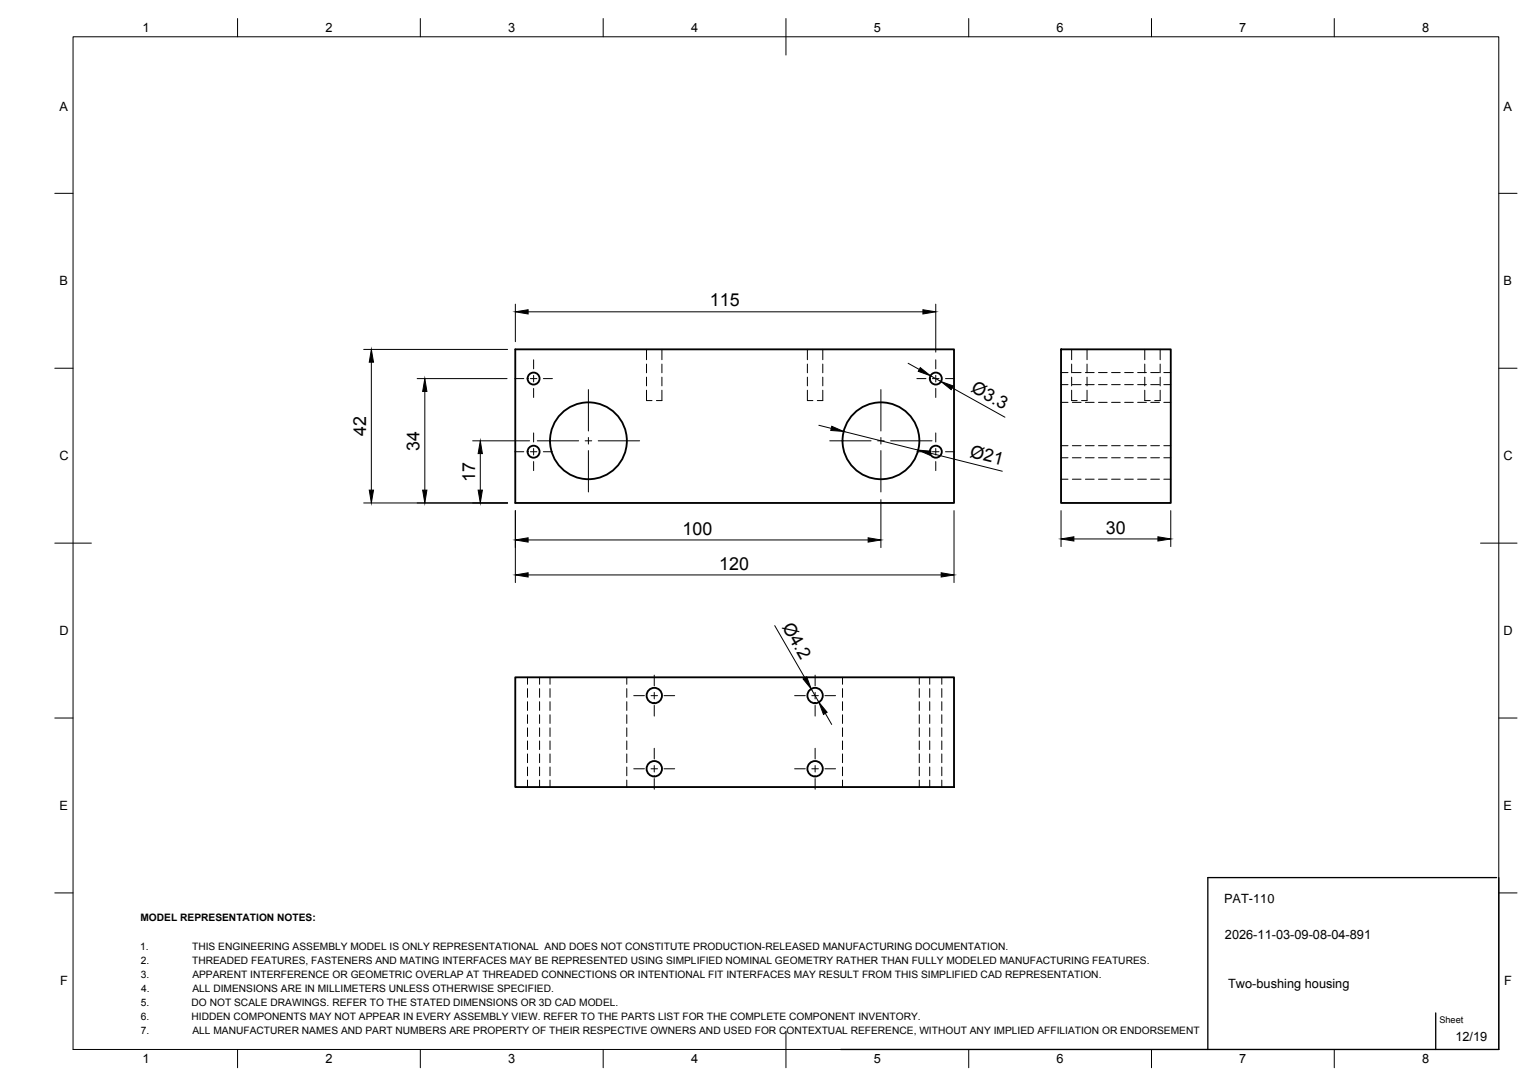
ISO-10303-21;
HEADER;
/* Generated by software containing ST-Developer
 * from STEP Tools, Inc. (www.steptools.com) 
 */

FILE_DESCRIPTION(
/* description */ ('Twin-shaft manual slide'),
/* implementation_level */ '2;1');

FILE_NAME(
/* name */ 'Two-bushing housing.step',
/* time_stamp */ '2026-10-27T18:38:08-07:00',
/* author */ (''),
/* organization */ (''),
/* preprocessor_version */ 'ST-DEVELOPER v20.2',
/* originating_system */ 'Autodesk Translation Framework v15.17.0.0',
/* authorisation */ '');

FILE_SCHEMA (('AUTOMOTIVE_DESIGN { 1 0 10303 214 3 1 1 }'));
ENDSEC;

DATA;
#10=MECHANICAL_DESIGN_GEOMETRIC_PRESENTATION_REPRESENTATION('',(#282),#6463);
#250=SHAPE_REPRESENTATION_RELATIONSHIP('SRR','None',#6569,#266);
#266=ADVANCED_BREP_SHAPE_REPRESENTATION('',(#297),#6452);
#282=STYLED_ITEM('',(#6719),#297);
#297=MANIFOLD_SOLID_BREP('Body1',#3645);
#345=FACE_BOUND('',#870,.T.);
#346=FACE_BOUND('',#871,.T.);
#347=FACE_BOUND('',#872,.T.);
#348=FACE_BOUND('',#873,.T.);
#349=FACE_BOUND('',#874,.T.);
#350=FACE_BOUND('',#875,.T.);
#351=FACE_BOUND('',#878,.T.);
#352=FACE_BOUND('',#879,.T.);
#353=FACE_BOUND('',#880,.T.);
#354=FACE_BOUND('',#881,.T.);
#355=FACE_BOUND('',#882,.T.);
#356=FACE_BOUND('',#883,.T.);
#357=FACE_BOUND('',#885,.T.);
#358=FACE_BOUND('',#886,.T.);
#359=FACE_BOUND('',#887,.T.);
#360=FACE_BOUND('',#888,.T.);
#450=PLANE('',#3997);
#451=PLANE('',#4001);
#452=PLANE('',#4005);
#453=PLANE('',#4009);
#454=PLANE('',#4016);
#455=PLANE('',#4017);
#456=PLANE('',#4018);
#457=PLANE('',#4019);
#458=PLANE('',#4020);
#459=PLANE('',#4021);
#606=FACE_OUTER_BOUND('',#854,.T.);
#607=FACE_OUTER_BOUND('',#855,.T.);
#608=FACE_OUTER_BOUND('',#856,.T.);
#609=FACE_OUTER_BOUND('',#857,.T.);
#610=FACE_OUTER_BOUND('',#858,.T.);
#611=FACE_OUTER_BOUND('',#859,.T.);
#612=FACE_OUTER_BOUND('',#860,.T.);
#613=FACE_OUTER_BOUND('',#861,.T.);
#614=FACE_OUTER_BOUND('',#862,.T.);
#615=FACE_OUTER_BOUND('',#863,.T.);
#616=FACE_OUTER_BOUND('',#864,.T.);
#617=FACE_OUTER_BOUND('',#865,.T.);
#618=FACE_OUTER_BOUND('',#866,.T.);
#619=FACE_OUTER_BOUND('',#867,.T.);
#620=FACE_OUTER_BOUND('',#868,.T.);
#621=FACE_OUTER_BOUND('',#869,.T.);
#622=FACE_OUTER_BOUND('',#876,.T.);
#623=FACE_OUTER_BOUND('',#877,.T.);
#624=FACE_OUTER_BOUND('',#884,.T.);
#625=FACE_OUTER_BOUND('',#889,.T.);
#854=EDGE_LOOP('',(#2856,#2857,#2858,#2859));
#855=EDGE_LOOP('',(#2860,#2861,#2862,#2863));
#856=EDGE_LOOP('',(#2864,#2865,#2866,#2867));
#857=EDGE_LOOP('',(#2868,#2869,#2870,#2871));
#858=EDGE_LOOP('',(#2872,#2873,#2874,#2875));
#859=EDGE_LOOP('',(#2876));
#860=EDGE_LOOP('',(#2877,#2878,#2879,#2880));
#861=EDGE_LOOP('',(#2881));
#862=EDGE_LOOP('',(#2882,#2883,#2884,#2885));
#863=EDGE_LOOP('',(#2886));
#864=EDGE_LOOP('',(#2887,#2888,#2889,#2890));
#865=EDGE_LOOP('',(#2891));
#866=EDGE_LOOP('',(#2892,#2893,#2894,#2895));
#867=EDGE_LOOP('',(#2896,#2897,#2898,#2899));
#868=EDGE_LOOP('',(#2900,#2901,#2902,#2903));
#869=EDGE_LOOP('',(#2904,#2905,#2906,#2907));
#870=EDGE_LOOP('',(#2908));
#871=EDGE_LOOP('',(#2909));
#872=EDGE_LOOP('',(#2910));
#873=EDGE_LOOP('',(#2911));
#874=EDGE_LOOP('',(#2912));
#875=EDGE_LOOP('',(#2913));
#876=EDGE_LOOP('',(#2914,#2915,#2916,#2917));
#877=EDGE_LOOP('',(#2918,#2919,#2920,#2921));
#878=EDGE_LOOP('',(#2922));
#879=EDGE_LOOP('',(#2923));
#880=EDGE_LOOP('',(#2924));
#881=EDGE_LOOP('',(#2925));
#882=EDGE_LOOP('',(#2926));
#883=EDGE_LOOP('',(#2927));
#884=EDGE_LOOP('',(#2928,#2929,#2930,#2931));
#885=EDGE_LOOP('',(#2932));
#886=EDGE_LOOP('',(#2933));
#887=EDGE_LOOP('',(#2934));
#888=EDGE_LOOP('',(#2935));
#889=EDGE_LOOP('',(#2936,#2937,#2938,#2939));
#1164=LINE('',#5816,#1450);
#1165=LINE('',#5822,#1451);
#1166=LINE('',#5828,#1452);
#1167=LINE('',#5834,#1453);
#1168=LINE('',#5840,#1454);
#1169=LINE('',#5847,#1455);
#1170=LINE('',#5854,#1456);
#1171=LINE('',#5861,#1457);
#1172=LINE('',#5868,#1458);
#1173=LINE('',#5874,#1459);
#1174=LINE('',#5879,#1460);
#1175=LINE('',#5881,#1461);
#1176=LINE('',#5883,#1462);
#1177=LINE('',#5884,#1463);
#1178=LINE('',#5887,#1464);
#1179=LINE('',#5889,#1465);
#1180=LINE('',#5890,#1466);
#1181=LINE('',#5893,#1467);
#1182=LINE('',#5895,#1468);
#1183=LINE('',#5896,#1469);
#1184=LINE('',#5898,#1470);
#1185=LINE('',#5899,#1471);
#1450=VECTOR('',#4692,0.165);
#1451=VECTOR('',#4699,0.165);
#1452=VECTOR('',#4706,0.165);
#1453=VECTOR('',#4713,0.165);
#1454=VECTOR('',#4720,0.210000000000001);
#1455=VECTOR('',#4729,0.210000000000001);
#1456=VECTOR('',#4738,0.210000000000001);
#1457=VECTOR('',#4747,0.210000000000001);
#1458=VECTOR('',#4756,1.05);
#1459=VECTOR('',#4763,1.05);
#1460=VECTOR('',#4768,1.);
#1461=VECTOR('',#4769,1.);
#1462=VECTOR('',#4770,1.);
#1463=VECTOR('',#4771,1.);
#1464=VECTOR('',#4774,1.);
#1465=VECTOR('',#4775,1.);
#1466=VECTOR('',#4776,1.);
#1467=VECTOR('',#4779,1.);
#1468=VECTOR('',#4780,1.);
#1469=VECTOR('',#4781,1.);
#1470=VECTOR('',#4784,1.);
#1471=VECTOR('',#4785,1.);
#1666=CIRCLE('',#3983,0.165);
#1667=CIRCLE('',#3984,0.165);
#1668=CIRCLE('',#3986,0.165);
#1669=CIRCLE('',#3987,0.165);
#1670=CIRCLE('',#3989,0.165);
#1671=CIRCLE('',#3990,0.165);
#1672=CIRCLE('',#3992,0.165);
#1673=CIRCLE('',#3993,0.165);
#1674=CIRCLE('',#3995,0.210000000000001);
#1675=CIRCLE('',#3996,0.210000000000001);
#1676=CIRCLE('',#3999,0.210000000000001);
#1677=CIRCLE('',#4000,0.210000000000001);
#1678=CIRCLE('',#4003,0.210000000000001);
#1679=CIRCLE('',#4004,0.210000000000001);
#1680=CIRCLE('',#4007,0.210000000000001);
#1681=CIRCLE('',#4008,0.210000000000001);
#1682=CIRCLE('',#4011,1.05);
#1683=CIRCLE('',#4012,1.05);
#1684=CIRCLE('',#4014,1.05);
#1685=CIRCLE('',#4015,1.05);
#1883=VERTEX_POINT('',#5813);
#1884=VERTEX_POINT('',#5815);
#1885=VERTEX_POINT('',#5819);
#1886=VERTEX_POINT('',#5821);
#1887=VERTEX_POINT('',#5825);
#1888=VERTEX_POINT('',#5827);
#1889=VERTEX_POINT('',#5831);
#1890=VERTEX_POINT('',#5833);
#1891=VERTEX_POINT('',#5837);
#1892=VERTEX_POINT('',#5839);
#1893=VERTEX_POINT('',#5844);
#1894=VERTEX_POINT('',#5846);
#1895=VERTEX_POINT('',#5851);
#1896=VERTEX_POINT('',#5853);
#1897=VERTEX_POINT('',#5858);
#1898=VERTEX_POINT('',#5860);
#1899=VERTEX_POINT('',#5865);
#1900=VERTEX_POINT('',#5867);
#1901=VERTEX_POINT('',#5871);
#1902=VERTEX_POINT('',#5873);
#1903=VERTEX_POINT('',#5877);
#1904=VERTEX_POINT('',#5878);
#1905=VERTEX_POINT('',#5880);
#1906=VERTEX_POINT('',#5882);
#1907=VERTEX_POINT('',#5886);
#1908=VERTEX_POINT('',#5888);
#1909=VERTEX_POINT('',#5892);
#1910=VERTEX_POINT('',#5894);
#2233=EDGE_CURVE('',#1883,#1883,#1666,.T.);
#2234=EDGE_CURVE('',#1883,#1884,#1164,.T.);
#2235=EDGE_CURVE('',#1884,#1884,#1667,.T.);
#2236=EDGE_CURVE('',#1885,#1885,#1668,.T.);
#2237=EDGE_CURVE('',#1885,#1886,#1165,.T.);
#2238=EDGE_CURVE('',#1886,#1886,#1669,.T.);
#2239=EDGE_CURVE('',#1887,#1887,#1670,.T.);
#2240=EDGE_CURVE('',#1887,#1888,#1166,.T.);
#2241=EDGE_CURVE('',#1888,#1888,#1671,.T.);
#2242=EDGE_CURVE('',#1889,#1889,#1672,.T.);
#2243=EDGE_CURVE('',#1889,#1890,#1167,.T.);
#2244=EDGE_CURVE('',#1890,#1890,#1673,.T.);
#2245=EDGE_CURVE('',#1891,#1891,#1674,.T.);
#2246=EDGE_CURVE('',#1891,#1892,#1168,.T.);
#2247=EDGE_CURVE('',#1892,#1892,#1675,.T.);
#2248=EDGE_CURVE('',#1893,#1893,#1676,.T.);
#2249=EDGE_CURVE('',#1893,#1894,#1169,.T.);
#2250=EDGE_CURVE('',#1894,#1894,#1677,.T.);
#2251=EDGE_CURVE('',#1895,#1895,#1678,.T.);
#2252=EDGE_CURVE('',#1895,#1896,#1170,.T.);
#2253=EDGE_CURVE('',#1896,#1896,#1679,.T.);
#2254=EDGE_CURVE('',#1897,#1897,#1680,.T.);
#2255=EDGE_CURVE('',#1897,#1898,#1171,.T.);
#2256=EDGE_CURVE('',#1898,#1898,#1681,.T.);
#2257=EDGE_CURVE('',#1899,#1899,#1682,.T.);
#2258=EDGE_CURVE('',#1899,#1900,#1172,.T.);
#2259=EDGE_CURVE('',#1900,#1900,#1683,.T.);
#2260=EDGE_CURVE('',#1901,#1901,#1684,.T.);
#2261=EDGE_CURVE('',#1901,#1902,#1173,.T.);
#2262=EDGE_CURVE('',#1902,#1902,#1685,.T.);
#2263=EDGE_CURVE('',#1903,#1904,#1174,.T.);
#2264=EDGE_CURVE('',#1904,#1905,#1175,.T.);
#2265=EDGE_CURVE('',#1906,#1905,#1176,.T.);
#2266=EDGE_CURVE('',#1903,#1906,#1177,.T.);
#2267=EDGE_CURVE('',#1907,#1903,#1178,.T.);
#2268=EDGE_CURVE('',#1908,#1906,#1179,.T.);
#2269=EDGE_CURVE('',#1907,#1908,#1180,.T.);
#2270=EDGE_CURVE('',#1909,#1907,#1181,.T.);
#2271=EDGE_CURVE('',#1910,#1908,#1182,.T.);
#2272=EDGE_CURVE('',#1909,#1910,#1183,.T.);
#2273=EDGE_CURVE('',#1904,#1909,#1184,.T.);
#2274=EDGE_CURVE('',#1905,#1910,#1185,.T.);
#2856=ORIENTED_EDGE('',*,*,#2233,.F.);
#2857=ORIENTED_EDGE('',*,*,#2234,.T.);
#2858=ORIENTED_EDGE('',*,*,#2235,.F.);
#2859=ORIENTED_EDGE('',*,*,#2234,.F.);
#2860=ORIENTED_EDGE('',*,*,#2236,.F.);
#2861=ORIENTED_EDGE('',*,*,#2237,.T.);
#2862=ORIENTED_EDGE('',*,*,#2238,.F.);
#2863=ORIENTED_EDGE('',*,*,#2237,.F.);
#2864=ORIENTED_EDGE('',*,*,#2239,.F.);
#2865=ORIENTED_EDGE('',*,*,#2240,.T.);
#2866=ORIENTED_EDGE('',*,*,#2241,.F.);
#2867=ORIENTED_EDGE('',*,*,#2240,.F.);
#2868=ORIENTED_EDGE('',*,*,#2242,.F.);
#2869=ORIENTED_EDGE('',*,*,#2243,.T.);
#2870=ORIENTED_EDGE('',*,*,#2244,.F.);
#2871=ORIENTED_EDGE('',*,*,#2243,.F.);
#2872=ORIENTED_EDGE('',*,*,#2245,.F.);
#2873=ORIENTED_EDGE('',*,*,#2246,.T.);
#2874=ORIENTED_EDGE('',*,*,#2247,.F.);
#2875=ORIENTED_EDGE('',*,*,#2246,.F.);
#2876=ORIENTED_EDGE('',*,*,#2245,.T.);
#2877=ORIENTED_EDGE('',*,*,#2248,.F.);
#2878=ORIENTED_EDGE('',*,*,#2249,.T.);
#2879=ORIENTED_EDGE('',*,*,#2250,.F.);
#2880=ORIENTED_EDGE('',*,*,#2249,.F.);
#2881=ORIENTED_EDGE('',*,*,#2248,.T.);
#2882=ORIENTED_EDGE('',*,*,#2251,.F.);
#2883=ORIENTED_EDGE('',*,*,#2252,.T.);
#2884=ORIENTED_EDGE('',*,*,#2253,.F.);
#2885=ORIENTED_EDGE('',*,*,#2252,.F.);
#2886=ORIENTED_EDGE('',*,*,#2251,.T.);
#2887=ORIENTED_EDGE('',*,*,#2254,.F.);
#2888=ORIENTED_EDGE('',*,*,#2255,.T.);
#2889=ORIENTED_EDGE('',*,*,#2256,.F.);
#2890=ORIENTED_EDGE('',*,*,#2255,.F.);
#2891=ORIENTED_EDGE('',*,*,#2254,.T.);
#2892=ORIENTED_EDGE('',*,*,#2257,.F.);
#2893=ORIENTED_EDGE('',*,*,#2258,.T.);
#2894=ORIENTED_EDGE('',*,*,#2259,.F.);
#2895=ORIENTED_EDGE('',*,*,#2258,.F.);
#2896=ORIENTED_EDGE('',*,*,#2260,.F.);
#2897=ORIENTED_EDGE('',*,*,#2261,.T.);
#2898=ORIENTED_EDGE('',*,*,#2262,.F.);
#2899=ORIENTED_EDGE('',*,*,#2261,.F.);
#2900=ORIENTED_EDGE('',*,*,#2263,.T.);
#2901=ORIENTED_EDGE('',*,*,#2264,.T.);
#2902=ORIENTED_EDGE('',*,*,#2265,.F.);
#2903=ORIENTED_EDGE('',*,*,#2266,.F.);
#2904=ORIENTED_EDGE('',*,*,#2267,.T.);
#2905=ORIENTED_EDGE('',*,*,#2266,.T.);
#2906=ORIENTED_EDGE('',*,*,#2268,.F.);
#2907=ORIENTED_EDGE('',*,*,#2269,.F.);
#2908=ORIENTED_EDGE('',*,*,#2262,.T.);
#2909=ORIENTED_EDGE('',*,*,#2259,.T.);
#2910=ORIENTED_EDGE('',*,*,#2244,.T.);
#2911=ORIENTED_EDGE('',*,*,#2241,.T.);
#2912=ORIENTED_EDGE('',*,*,#2238,.T.);
#2913=ORIENTED_EDGE('',*,*,#2235,.T.);
#2914=ORIENTED_EDGE('',*,*,#2270,.T.);
#2915=ORIENTED_EDGE('',*,*,#2269,.T.);
#2916=ORIENTED_EDGE('',*,*,#2271,.F.);
#2917=ORIENTED_EDGE('',*,*,#2272,.F.);
#2918=ORIENTED_EDGE('',*,*,#2273,.T.);
#2919=ORIENTED_EDGE('',*,*,#2272,.T.);
#2920=ORIENTED_EDGE('',*,*,#2274,.F.);
#2921=ORIENTED_EDGE('',*,*,#2264,.F.);
#2922=ORIENTED_EDGE('',*,*,#2260,.T.);
#2923=ORIENTED_EDGE('',*,*,#2257,.T.);
#2924=ORIENTED_EDGE('',*,*,#2242,.T.);
#2925=ORIENTED_EDGE('',*,*,#2239,.T.);
#2926=ORIENTED_EDGE('',*,*,#2236,.T.);
#2927=ORIENTED_EDGE('',*,*,#2233,.T.);
#2928=ORIENTED_EDGE('',*,*,#2274,.T.);
#2929=ORIENTED_EDGE('',*,*,#2271,.T.);
#2930=ORIENTED_EDGE('',*,*,#2268,.T.);
#2931=ORIENTED_EDGE('',*,*,#2265,.T.);
#2932=ORIENTED_EDGE('',*,*,#2247,.T.);
#2933=ORIENTED_EDGE('',*,*,#2250,.T.);
#2934=ORIENTED_EDGE('',*,*,#2253,.T.);
#2935=ORIENTED_EDGE('',*,*,#2256,.T.);
#2936=ORIENTED_EDGE('',*,*,#2273,.F.);
#2937=ORIENTED_EDGE('',*,*,#2263,.F.);
#2938=ORIENTED_EDGE('',*,*,#2267,.F.);
#2939=ORIENTED_EDGE('',*,*,#2270,.F.);
#3392=CYLINDRICAL_SURFACE('',#3982,0.165);
#3393=CYLINDRICAL_SURFACE('',#3985,0.165);
#3394=CYLINDRICAL_SURFACE('',#3988,0.165);
#3395=CYLINDRICAL_SURFACE('',#3991,0.165);
#3396=CYLINDRICAL_SURFACE('',#3994,0.210000000000001);
#3397=CYLINDRICAL_SURFACE('',#3998,0.210000000000001);
#3398=CYLINDRICAL_SURFACE('',#4002,0.210000000000001);
#3399=CYLINDRICAL_SURFACE('',#4006,0.210000000000001);
#3400=CYLINDRICAL_SURFACE('',#4010,1.05);
#3401=CYLINDRICAL_SURFACE('',#4013,1.05);
#3511=ADVANCED_FACE('',(#606),#3392,.F.);
#3512=ADVANCED_FACE('',(#607),#3393,.F.);
#3513=ADVANCED_FACE('',(#608),#3394,.F.);
#3514=ADVANCED_FACE('',(#609),#3395,.F.);
#3515=ADVANCED_FACE('',(#610),#3396,.F.);
#3516=ADVANCED_FACE('',(#611),#450,.T.);
#3517=ADVANCED_FACE('',(#612),#3397,.F.);
#3518=ADVANCED_FACE('',(#613),#451,.T.);
#3519=ADVANCED_FACE('',(#614),#3398,.F.);
#3520=ADVANCED_FACE('',(#615),#452,.T.);
#3521=ADVANCED_FACE('',(#616),#3399,.F.);
#3522=ADVANCED_FACE('',(#617),#453,.T.);
#3523=ADVANCED_FACE('',(#618),#3400,.F.);
#3524=ADVANCED_FACE('',(#619),#3401,.F.);
#3525=ADVANCED_FACE('',(#620),#454,.T.);
#3526=ADVANCED_FACE('',(#621,#345,#346,#347,#348,#349,#350),#455,.T.);
#3527=ADVANCED_FACE('',(#622),#456,.T.);
#3528=ADVANCED_FACE('',(#623,#351,#352,#353,#354,#355,#356),#457,.T.);
#3529=ADVANCED_FACE('',(#624,#357,#358,#359,#360),#458,.T.);
#3530=ADVANCED_FACE('',(#625),#459,.F.);
#3645=CLOSED_SHELL('',(#3511,#3512,#3513,#3514,#3515,#3516,#3517,#3518,
#3519,#3520,#3521,#3522,#3523,#3524,#3525,#3526,#3527,#3528,#3529,#3530));
#3981=AXIS2_PLACEMENT_3D('',#5811,#4686,#4687);
#3982=AXIS2_PLACEMENT_3D('',#5812,#4688,#4689);
#3983=AXIS2_PLACEMENT_3D('',#5814,#4690,#4691);
#3984=AXIS2_PLACEMENT_3D('',#5817,#4693,#4694);
#3985=AXIS2_PLACEMENT_3D('',#5818,#4695,#4696);
#3986=AXIS2_PLACEMENT_3D('',#5820,#4697,#4698);
#3987=AXIS2_PLACEMENT_3D('',#5823,#4700,#4701);
#3988=AXIS2_PLACEMENT_3D('',#5824,#4702,#4703);
#3989=AXIS2_PLACEMENT_3D('',#5826,#4704,#4705);
#3990=AXIS2_PLACEMENT_3D('',#5829,#4707,#4708);
#3991=AXIS2_PLACEMENT_3D('',#5830,#4709,#4710);
#3992=AXIS2_PLACEMENT_3D('',#5832,#4711,#4712);
#3993=AXIS2_PLACEMENT_3D('',#5835,#4714,#4715);
#3994=AXIS2_PLACEMENT_3D('',#5836,#4716,#4717);
#3995=AXIS2_PLACEMENT_3D('',#5838,#4718,#4719);
#3996=AXIS2_PLACEMENT_3D('',#5841,#4721,#4722);
#3997=AXIS2_PLACEMENT_3D('',#5842,#4723,#4724);
#3998=AXIS2_PLACEMENT_3D('',#5843,#4725,#4726);
#3999=AXIS2_PLACEMENT_3D('',#5845,#4727,#4728);
#4000=AXIS2_PLACEMENT_3D('',#5848,#4730,#4731);
#4001=AXIS2_PLACEMENT_3D('',#5849,#4732,#4733);
#4002=AXIS2_PLACEMENT_3D('',#5850,#4734,#4735);
#4003=AXIS2_PLACEMENT_3D('',#5852,#4736,#4737);
#4004=AXIS2_PLACEMENT_3D('',#5855,#4739,#4740);
#4005=AXIS2_PLACEMENT_3D('',#5856,#4741,#4742);
#4006=AXIS2_PLACEMENT_3D('',#5857,#4743,#4744);
#4007=AXIS2_PLACEMENT_3D('',#5859,#4745,#4746);
#4008=AXIS2_PLACEMENT_3D('',#5862,#4748,#4749);
#4009=AXIS2_PLACEMENT_3D('',#5863,#4750,#4751);
#4010=AXIS2_PLACEMENT_3D('',#5864,#4752,#4753);
#4011=AXIS2_PLACEMENT_3D('',#5866,#4754,#4755);
#4012=AXIS2_PLACEMENT_3D('',#5869,#4757,#4758);
#4013=AXIS2_PLACEMENT_3D('',#5870,#4759,#4760);
#4014=AXIS2_PLACEMENT_3D('',#5872,#4761,#4762);
#4015=AXIS2_PLACEMENT_3D('',#5875,#4764,#4765);
#4016=AXIS2_PLACEMENT_3D('',#5876,#4766,#4767);
#4017=AXIS2_PLACEMENT_3D('',#5885,#4772,#4773);
#4018=AXIS2_PLACEMENT_3D('',#5891,#4777,#4778);
#4019=AXIS2_PLACEMENT_3D('',#5897,#4782,#4783);
#4020=AXIS2_PLACEMENT_3D('',#5900,#4786,#4787);
#4021=AXIS2_PLACEMENT_3D('',#5901,#4788,#4789);
#4686=DIRECTION('axis',(0.,0.,1.));
#4687=DIRECTION('refdir',(1.,0.,0.));
#4688=DIRECTION('center_axis',(1.,0.,0.));
#4689=DIRECTION('ref_axis',(0.,0.,-1.));
#4690=DIRECTION('center_axis',(1.,0.,0.));
#4691=DIRECTION('ref_axis',(0.,0.,-1.));
#4692=DIRECTION('',(1.,0.,0.));
#4693=DIRECTION('center_axis',(-1.,0.,0.));
#4694=DIRECTION('ref_axis',(0.,0.,-1.));
#4695=DIRECTION('center_axis',(1.,0.,0.));
#4696=DIRECTION('ref_axis',(0.,0.,-1.));
#4697=DIRECTION('center_axis',(1.,0.,0.));
#4698=DIRECTION('ref_axis',(0.,0.,-1.));
#4699=DIRECTION('',(1.,0.,0.));
#4700=DIRECTION('center_axis',(-1.,0.,0.));
#4701=DIRECTION('ref_axis',(0.,0.,-1.));
#4702=DIRECTION('center_axis',(1.,0.,0.));
#4703=DIRECTION('ref_axis',(0.,0.,-1.));
#4704=DIRECTION('center_axis',(1.,0.,0.));
#4705=DIRECTION('ref_axis',(0.,0.,-1.));
#4706=DIRECTION('',(1.,0.,0.));
#4707=DIRECTION('center_axis',(-1.,0.,0.));
#4708=DIRECTION('ref_axis',(0.,0.,-1.));
#4709=DIRECTION('center_axis',(1.,0.,0.));
#4710=DIRECTION('ref_axis',(0.,0.,-1.));
#4711=DIRECTION('center_axis',(1.,0.,0.));
#4712=DIRECTION('ref_axis',(0.,0.,-1.));
#4713=DIRECTION('',(1.,0.,0.));
#4714=DIRECTION('center_axis',(-1.,0.,0.));
#4715=DIRECTION('ref_axis',(0.,0.,-1.));
#4716=DIRECTION('center_axis',(0.,0.,1.));
#4717=DIRECTION('ref_axis',(1.,0.,0.));
#4718=DIRECTION('center_axis',(0.,0.,1.));
#4719=DIRECTION('ref_axis',(1.,0.,0.));
#4720=DIRECTION('',(0.,0.,1.));
#4721=DIRECTION('center_axis',(0.,0.,-1.));
#4722=DIRECTION('ref_axis',(1.,0.,0.));
#4723=DIRECTION('center_axis',(0.,0.,1.));
#4724=DIRECTION('ref_axis',(1.,0.,0.));
#4725=DIRECTION('center_axis',(0.,0.,1.));
#4726=DIRECTION('ref_axis',(1.,0.,0.));
#4727=DIRECTION('center_axis',(0.,0.,1.));
#4728=DIRECTION('ref_axis',(1.,0.,0.));
#4729=DIRECTION('',(0.,0.,1.));
#4730=DIRECTION('center_axis',(0.,0.,-1.));
#4731=DIRECTION('ref_axis',(1.,0.,0.));
#4732=DIRECTION('center_axis',(0.,0.,1.));
#4733=DIRECTION('ref_axis',(1.,0.,0.));
#4734=DIRECTION('center_axis',(0.,0.,1.));
#4735=DIRECTION('ref_axis',(1.,0.,0.));
#4736=DIRECTION('center_axis',(0.,0.,1.));
#4737=DIRECTION('ref_axis',(1.,0.,0.));
#4738=DIRECTION('',(0.,0.,1.));
#4739=DIRECTION('center_axis',(0.,0.,-1.));
#4740=DIRECTION('ref_axis',(1.,0.,0.));
#4741=DIRECTION('center_axis',(0.,0.,1.));
#4742=DIRECTION('ref_axis',(1.,0.,0.));
#4743=DIRECTION('center_axis',(0.,0.,1.));
#4744=DIRECTION('ref_axis',(1.,0.,0.));
#4745=DIRECTION('center_axis',(0.,0.,1.));
#4746=DIRECTION('ref_axis',(1.,0.,0.));
#4747=DIRECTION('',(0.,0.,1.));
#4748=DIRECTION('center_axis',(0.,0.,-1.));
#4749=DIRECTION('ref_axis',(1.,0.,0.));
#4750=DIRECTION('center_axis',(0.,0.,1.));
#4751=DIRECTION('ref_axis',(1.,0.,0.));
#4752=DIRECTION('center_axis',(1.,0.,0.));
#4753=DIRECTION('ref_axis',(0.,0.,-1.));
#4754=DIRECTION('center_axis',(1.,0.,0.));
#4755=DIRECTION('ref_axis',(0.,0.,-1.));
#4756=DIRECTION('',(1.,0.,0.));
#4757=DIRECTION('center_axis',(-1.,0.,0.));
#4758=DIRECTION('ref_axis',(0.,0.,-1.));
#4759=DIRECTION('center_axis',(1.,0.,0.));
#4760=DIRECTION('ref_axis',(0.,0.,-1.));
#4761=DIRECTION('center_axis',(1.,0.,0.));
#4762=DIRECTION('ref_axis',(0.,0.,-1.));
#4763=DIRECTION('',(1.,0.,0.));
#4764=DIRECTION('center_axis',(-1.,0.,0.));
#4765=DIRECTION('ref_axis',(0.,0.,-1.));
#4766=DIRECTION('center_axis',(0.,1.,0.));
#4767=DIRECTION('ref_axis',(-1.,0.,0.));
#4768=DIRECTION('',(-1.,0.,0.));
#4769=DIRECTION('',(0.,0.,1.));
#4770=DIRECTION('',(-1.,0.,0.));
#4771=DIRECTION('',(0.,0.,1.));
#4772=DIRECTION('center_axis',(1.,0.,0.));
#4773=DIRECTION('ref_axis',(0.,1.,0.));
#4774=DIRECTION('',(0.,1.,0.));
#4775=DIRECTION('',(0.,1.,0.));
#4776=DIRECTION('',(0.,0.,1.));
#4777=DIRECTION('center_axis',(0.,-1.,0.));
#4778=DIRECTION('ref_axis',(1.,0.,0.));
#4779=DIRECTION('',(1.,0.,0.));
#4780=DIRECTION('',(1.,0.,0.));
#4781=DIRECTION('',(0.,0.,1.));
#4782=DIRECTION('center_axis',(-1.,0.,0.));
#4783=DIRECTION('ref_axis',(0.,-1.,0.));
#4784=DIRECTION('',(0.,-1.,0.));
#4785=DIRECTION('',(0.,-1.,0.));
#4786=DIRECTION('center_axis',(0.,0.,1.));
#4787=DIRECTION('ref_axis',(1.,0.,0.));
#4788=DIRECTION('center_axis',(0.,0.,1.));
#4789=DIRECTION('ref_axis',(1.,0.,0.));
#5811=CARTESIAN_POINT('',(0.,0.,0.));
#5812=CARTESIAN_POINT('Origin',(13.4,5.5,3.));
#5813=CARTESIAN_POINT('',(13.5,5.5,3.165));
#5814=CARTESIAN_POINT('Origin',(13.5,5.5,3.));
#5815=CARTESIAN_POINT('',(16.5,5.5,3.165));
#5816=CARTESIAN_POINT('',(13.4,5.5,3.165));
#5817=CARTESIAN_POINT('Origin',(16.5,5.5,3.));
#5818=CARTESIAN_POINT('Origin',(13.4,-5.5,5.));
#5819=CARTESIAN_POINT('',(13.5,-5.5,5.165));
#5820=CARTESIAN_POINT('Origin',(13.5,-5.5,5.));
#5821=CARTESIAN_POINT('',(16.5,-5.5,5.165));
#5822=CARTESIAN_POINT('',(13.4,-5.5,5.165));
#5823=CARTESIAN_POINT('Origin',(16.5,-5.5,5.));
#5824=CARTESIAN_POINT('Origin',(13.4,-5.5,3.));
#5825=CARTESIAN_POINT('',(13.5,-5.5,3.165));
#5826=CARTESIAN_POINT('Origin',(13.5,-5.5,3.));
#5827=CARTESIAN_POINT('',(16.5,-5.5,3.165));
#5828=CARTESIAN_POINT('',(13.4,-5.5,3.165));
#5829=CARTESIAN_POINT('Origin',(16.5,-5.5,3.));
#5830=CARTESIAN_POINT('Origin',(13.4,5.5,5.));
#5831=CARTESIAN_POINT('',(13.5,5.5,5.165));
#5832=CARTESIAN_POINT('Origin',(13.5,5.5,5.));
#5833=CARTESIAN_POINT('',(16.5,5.5,5.165));
#5834=CARTESIAN_POINT('',(13.4,5.5,5.165));
#5835=CARTESIAN_POINT('Origin',(16.5,5.5,5.));
#5836=CARTESIAN_POINT('Origin',(16.,-2.2,4.4));
#5837=CARTESIAN_POINT('',(15.79,-2.2,4.4));
#5838=CARTESIAN_POINT('Origin',(16.,-2.2,4.4));
#5839=CARTESIAN_POINT('',(15.79,-2.2,5.8));
#5840=CARTESIAN_POINT('',(15.79,-2.2,4.4));
#5841=CARTESIAN_POINT('Origin',(16.,-2.2,5.8));
#5842=CARTESIAN_POINT('Origin',(16.,-2.2,4.4));
#5843=CARTESIAN_POINT('Origin',(14.,2.2,4.4));
#5844=CARTESIAN_POINT('',(13.79,2.2,4.4));
#5845=CARTESIAN_POINT('Origin',(14.,2.2,4.4));
#5846=CARTESIAN_POINT('',(13.79,2.2,5.8));
#5847=CARTESIAN_POINT('',(13.79,2.2,4.4));
#5848=CARTESIAN_POINT('Origin',(14.,2.2,5.8));
#5849=CARTESIAN_POINT('Origin',(14.,2.2,4.4));
#5850=CARTESIAN_POINT('Origin',(14.,-2.2,4.4));
#5851=CARTESIAN_POINT('',(13.79,-2.2,4.4));
#5852=CARTESIAN_POINT('Origin',(14.,-2.2,4.4));
#5853=CARTESIAN_POINT('',(13.79,-2.2,5.8));
#5854=CARTESIAN_POINT('',(13.79,-2.2,4.4));
#5855=CARTESIAN_POINT('Origin',(14.,-2.2,5.8));
#5856=CARTESIAN_POINT('Origin',(14.,-2.2,4.4));
#5857=CARTESIAN_POINT('Origin',(16.,2.2,4.4));
#5858=CARTESIAN_POINT('',(15.79,2.2,4.4));
#5859=CARTESIAN_POINT('Origin',(16.,2.2,4.4));
#5860=CARTESIAN_POINT('',(15.79,2.2,5.8));
#5861=CARTESIAN_POINT('',(15.79,2.2,4.4));
#5862=CARTESIAN_POINT('Origin',(16.,2.2,5.8));
#5863=CARTESIAN_POINT('Origin',(16.,2.2,4.4));
#5864=CARTESIAN_POINT('Origin',(13.4,-4.,3.3));
#5865=CARTESIAN_POINT('',(13.5,-4.,4.35));
#5866=CARTESIAN_POINT('Origin',(13.5,-4.,3.3));
#5867=CARTESIAN_POINT('',(16.5,-4.,4.35));
#5868=CARTESIAN_POINT('',(13.4,-4.,4.35));
#5869=CARTESIAN_POINT('Origin',(16.5,-4.,3.3));
#5870=CARTESIAN_POINT('Origin',(13.4,4.,3.3));
#5871=CARTESIAN_POINT('',(13.5,4.,4.35));
#5872=CARTESIAN_POINT('Origin',(13.5,4.,3.3));
#5873=CARTESIAN_POINT('',(16.5,4.,4.35));
#5874=CARTESIAN_POINT('',(13.4,4.,4.35));
#5875=CARTESIAN_POINT('Origin',(16.5,4.,3.3));
#5876=CARTESIAN_POINT('Origin',(16.5,6.,1.6));
#5877=CARTESIAN_POINT('',(16.5,6.,1.6));
#5878=CARTESIAN_POINT('',(13.5,6.,1.6));
#5879=CARTESIAN_POINT('',(16.5,6.,1.6));
#5880=CARTESIAN_POINT('',(13.5,6.,5.8));
#5881=CARTESIAN_POINT('',(13.5,6.,1.6));
#5882=CARTESIAN_POINT('',(16.5,6.,5.8));
#5883=CARTESIAN_POINT('',(16.5,6.,5.8));
#5884=CARTESIAN_POINT('',(16.5,6.,1.6));
#5885=CARTESIAN_POINT('Origin',(16.5,-6.,1.6));
#5886=CARTESIAN_POINT('',(16.5,-6.,1.6));
#5887=CARTESIAN_POINT('',(16.5,-6.,1.6));
#5888=CARTESIAN_POINT('',(16.5,-6.,5.8));
#5889=CARTESIAN_POINT('',(16.5,-6.,5.8));
#5890=CARTESIAN_POINT('',(16.5,-6.,1.6));
#5891=CARTESIAN_POINT('Origin',(13.5,-6.,1.6));
#5892=CARTESIAN_POINT('',(13.5,-6.,1.6));
#5893=CARTESIAN_POINT('',(13.5,-6.,1.6));
#5894=CARTESIAN_POINT('',(13.5,-6.,5.8));
#5895=CARTESIAN_POINT('',(13.5,-6.,5.8));
#5896=CARTESIAN_POINT('',(13.5,-6.,1.6));
#5897=CARTESIAN_POINT('Origin',(13.5,6.,1.6));
#5898=CARTESIAN_POINT('',(13.5,6.,1.6));
#5899=CARTESIAN_POINT('',(13.5,6.,5.8));
#5900=CARTESIAN_POINT('Origin',(15.,0.,5.8));
#5901=CARTESIAN_POINT('Origin',(15.,0.,1.6));
#6431=UNCERTAINTY_MEASURE_WITH_UNIT(LENGTH_MEASURE(0.001),#6464,
'DISTANCE_ACCURACY_VALUE',
'Maximum model space distance between geometric entities at asserted c
onnectivities');
#6442=UNCERTAINTY_MEASURE_WITH_UNIT(LENGTH_MEASURE(0.001),#6464,
'DISTANCE_ACCURACY_VALUE',
'Maximum model space distance between geometric entities at asserted c
onnectivities');
#6452=(
GEOMETRIC_REPRESENTATION_CONTEXT(3)
GLOBAL_UNCERTAINTY_ASSIGNED_CONTEXT((#6431))
GLOBAL_UNIT_ASSIGNED_CONTEXT((#6464,#6466,#6467))
REPRESENTATION_CONTEXT('','3D')
);
#6463=(
GEOMETRIC_REPRESENTATION_CONTEXT(3)
GLOBAL_UNCERTAINTY_ASSIGNED_CONTEXT((#6442))
GLOBAL_UNIT_ASSIGNED_CONTEXT((#6464,#6466,#6467))
REPRESENTATION_CONTEXT('','3D')
);
#6464=(
LENGTH_UNIT()
NAMED_UNIT(*)
SI_UNIT(.CENTI.,.METRE.)
);
#6466=(
NAMED_UNIT(*)
PLANE_ANGLE_UNIT()
SI_UNIT($,.RADIAN.)
);
#6467=(
NAMED_UNIT(*)
SI_UNIT($,.STERADIAN.)
SOLID_ANGLE_UNIT()
);
#6477=SHAPE_DEFINITION_REPRESENTATION(#6497,#6569);
#6497=PRODUCT_DEFINITION_SHAPE('',$,#6590);
#6569=SHAPE_REPRESENTATION('',(#3981),#6452);
#6580=PRODUCT_DEFINITION_CONTEXT('part definition',#6642,'design');
#6590=PRODUCT_DEFINITION('Two-bushing housing','Two-bushing housing',#6610,
#6580);
#6610=PRODUCT_DEFINITION_FORMATION('',$,#6653);
#6642=APPLICATION_CONTEXT(
'Core Data for Automotive Mechanical Design Process');
#6643=PRODUCT_CONTEXT('part definition',#6642,'mechanical');
#6653=PRODUCT('Two-bushing housing','Two-bushing housing',
'Two-bushing housing',(#6643));
#6713=COLOUR_RGB('Dark Blue',0.08,0.2,0.34);
#6714=FILL_AREA_STYLE_COLOUR('',#6713);
#6715=FILL_AREA_STYLE('',(#6714));
#6716=SURFACE_STYLE_FILL_AREA(#6715);
#6717=SURFACE_SIDE_STYLE('',(#6716));
#6718=SURFACE_STYLE_USAGE(.BOTH.,#6717);
#6719=PRESENTATION_STYLE_ASSIGNMENT((#6718));
ENDSEC;
END-ISO-10303-21;
